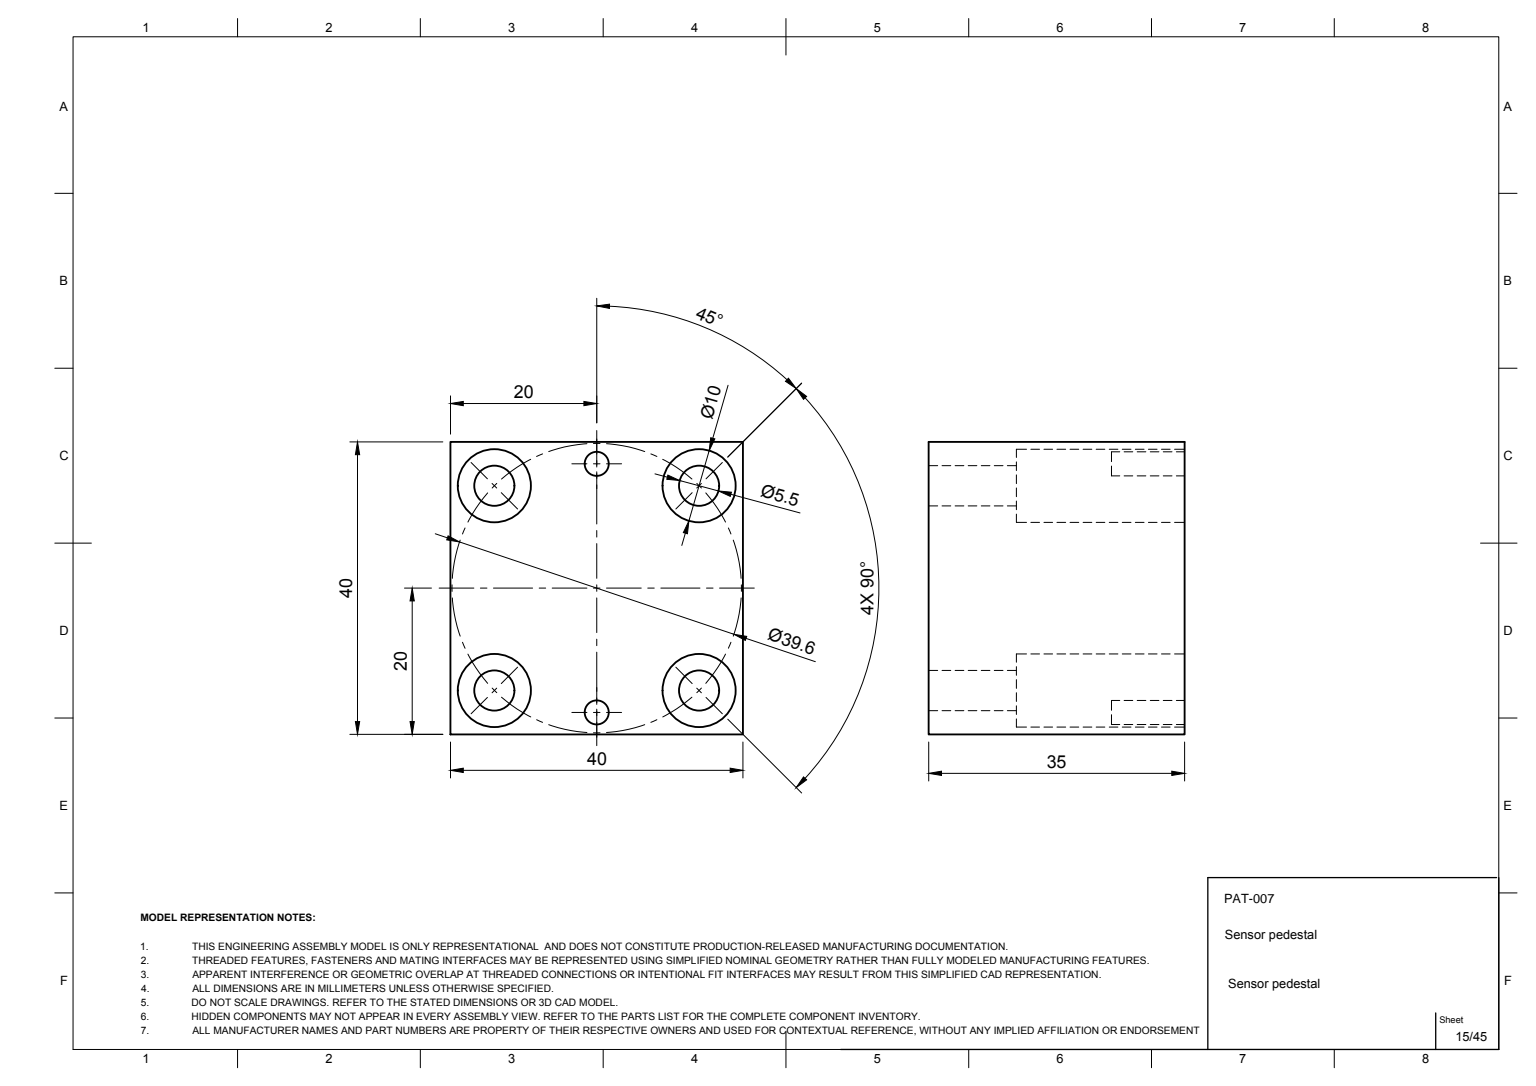
ISO-10303-21;
HEADER;
/* Generated by software containing ST-Developer
 * from STEP Tools, Inc. (www.steptools.com) 
 */

FILE_DESCRIPTION(
/* description */ ('Bearing friction torque test rig'),
/* implementation_level */ '2;1');

FILE_NAME(
/* name */ 'Sensor pedestal.step',
/* time_stamp */ '2026-10-28T03:24:04-07:00',
/* author */ (''),
/* organization */ (''),
/* preprocessor_version */ 'ST-DEVELOPER v20.2',
/* originating_system */ 'Autodesk Translation Framework v15.17.0.0',
/* authorisation */ '');

FILE_SCHEMA (('AUTOMOTIVE_DESIGN { 1 0 10303 214 3 1 1 }'));
ENDSEC;

DATA;
#10=MECHANICAL_DESIGN_GEOMETRIC_PRESENTATION_REPRESENTATION('',(#549),#14822);
#471=SHAPE_REPRESENTATION_RELATIONSHIP('SRR','None',#15010,#510);
#510=ADVANCED_BREP_SHAPE_REPRESENTATION('',(#603),#14790);
#549=STYLED_ITEM('',(#15298),#603);
#603=MANIFOLD_SOLID_BREP('Body1',#7665);
#777=FACE_BOUND('',#1816,.T.);
#778=FACE_BOUND('',#1819,.T.);
#779=FACE_BOUND('',#1822,.T.);
#780=FACE_BOUND('',#1825,.T.);
#781=FACE_BOUND('',#1835,.T.);
#782=FACE_BOUND('',#1836,.T.);
#783=FACE_BOUND('',#1837,.T.);
#784=FACE_BOUND('',#1838,.T.);
#785=FACE_BOUND('',#1839,.T.);
#786=FACE_BOUND('',#1840,.T.);
#787=FACE_BOUND('',#1842,.T.);
#788=FACE_BOUND('',#1843,.T.);
#789=FACE_BOUND('',#1844,.T.);
#790=FACE_BOUND('',#1845,.T.);
#927=PLANE('',#8461);
#928=PLANE('',#8465);
#929=PLANE('',#8469);
#930=PLANE('',#8474);
#931=PLANE('',#8479);
#932=PLANE('',#8484);
#933=PLANE('',#8494);
#934=PLANE('',#8495);
#935=PLANE('',#8496);
#936=PLANE('',#8497);
#937=PLANE('',#8498);
#938=PLANE('',#8499);
#1232=FACE_OUTER_BOUND('',#1810,.T.);
#1233=FACE_OUTER_BOUND('',#1811,.T.);
#1234=FACE_OUTER_BOUND('',#1812,.T.);
#1235=FACE_OUTER_BOUND('',#1813,.T.);
#1236=FACE_OUTER_BOUND('',#1814,.T.);
#1237=FACE_OUTER_BOUND('',#1815,.T.);
#1238=FACE_OUTER_BOUND('',#1817,.T.);
#1239=FACE_OUTER_BOUND('',#1818,.T.);
#1240=FACE_OUTER_BOUND('',#1820,.T.);
#1241=FACE_OUTER_BOUND('',#1821,.T.);
#1242=FACE_OUTER_BOUND('',#1823,.T.);
#1243=FACE_OUTER_BOUND('',#1824,.T.);
#1244=FACE_OUTER_BOUND('',#1826,.T.);
#1245=FACE_OUTER_BOUND('',#1827,.T.);
#1246=FACE_OUTER_BOUND('',#1828,.T.);
#1247=FACE_OUTER_BOUND('',#1829,.T.);
#1248=FACE_OUTER_BOUND('',#1830,.T.);
#1249=FACE_OUTER_BOUND('',#1831,.T.);
#1250=FACE_OUTER_BOUND('',#1832,.T.);
#1251=FACE_OUTER_BOUND('',#1833,.T.);
#1252=FACE_OUTER_BOUND('',#1834,.T.);
#1253=FACE_OUTER_BOUND('',#1841,.T.);
#1810=EDGE_LOOP('',(#5760,#5761,#5762,#5763));
#1811=EDGE_LOOP('',(#5764));
#1812=EDGE_LOOP('',(#5765,#5766,#5767,#5768));
#1813=EDGE_LOOP('',(#5769));
#1814=EDGE_LOOP('',(#5770,#5771,#5772,#5773));
#1815=EDGE_LOOP('',(#5774));
#1816=EDGE_LOOP('',(#5775));
#1817=EDGE_LOOP('',(#5776,#5777,#5778,#5779));
#1818=EDGE_LOOP('',(#5780));
#1819=EDGE_LOOP('',(#5781));
#1820=EDGE_LOOP('',(#5782,#5783,#5784,#5785));
#1821=EDGE_LOOP('',(#5786));
#1822=EDGE_LOOP('',(#5787));
#1823=EDGE_LOOP('',(#5788,#5789,#5790,#5791));
#1824=EDGE_LOOP('',(#5792));
#1825=EDGE_LOOP('',(#5793));
#1826=EDGE_LOOP('',(#5794,#5795,#5796,#5797));
#1827=EDGE_LOOP('',(#5798,#5799,#5800,#5801));
#1828=EDGE_LOOP('',(#5802,#5803,#5804,#5805));
#1829=EDGE_LOOP('',(#5806,#5807,#5808,#5809));
#1830=EDGE_LOOP('',(#5810,#5811,#5812,#5813));
#1831=EDGE_LOOP('',(#5814,#5815,#5816,#5817));
#1832=EDGE_LOOP('',(#5818,#5819,#5820,#5821));
#1833=EDGE_LOOP('',(#5822,#5823,#5824,#5825));
#1834=EDGE_LOOP('',(#5826,#5827,#5828,#5829));
#1835=EDGE_LOOP('',(#5830));
#1836=EDGE_LOOP('',(#5831));
#1837=EDGE_LOOP('',(#5832));
#1838=EDGE_LOOP('',(#5833));
#1839=EDGE_LOOP('',(#5834));
#1840=EDGE_LOOP('',(#5835));
#1841=EDGE_LOOP('',(#5836,#5837,#5838,#5839));
#1842=EDGE_LOOP('',(#5840));
#1843=EDGE_LOOP('',(#5841));
#1844=EDGE_LOOP('',(#5842));
#1845=EDGE_LOOP('',(#5843));
#2355=LINE('',#12318,#2799);
#2356=LINE('',#12325,#2800);
#2357=LINE('',#12332,#2801);
#2358=LINE('',#12341,#2802);
#2359=LINE('',#12350,#2803);
#2360=LINE('',#12359,#2804);
#2361=LINE('',#12367,#2805);
#2362=LINE('',#12371,#2806);
#2363=LINE('',#12375,#2807);
#2364=LINE('',#12379,#2808);
#2365=LINE('',#12383,#2809);
#2366=LINE('',#12385,#2810);
#2367=LINE('',#12387,#2811);
#2368=LINE('',#12388,#2812);
#2369=LINE('',#12391,#2813);
#2370=LINE('',#12393,#2814);
#2371=LINE('',#12394,#2815);
#2372=LINE('',#12397,#2816);
#2373=LINE('',#12399,#2817);
#2374=LINE('',#12400,#2818);
#2375=LINE('',#12402,#2819);
#2376=LINE('',#12403,#2820);
#2799=VECTOR('',#9938,0.164999999999999);
#2800=VECTOR('',#9947,0.164999999999999);
#2801=VECTOR('',#9956,0.5);
#2802=VECTOR('',#9967,0.5);
#2803=VECTOR('',#9978,0.5);
#2804=VECTOR('',#9989,0.5);
#2805=VECTOR('',#10000,0.275);
#2806=VECTOR('',#10005,0.275);
#2807=VECTOR('',#10010,0.275);
#2808=VECTOR('',#10015,0.275);
#2809=VECTOR('',#10018,1.);
#2810=VECTOR('',#10019,1.);
#2811=VECTOR('',#10020,1.);
#2812=VECTOR('',#10021,1.);
#2813=VECTOR('',#10024,1.);
#2814=VECTOR('',#10025,1.);
#2815=VECTOR('',#10026,1.);
#2816=VECTOR('',#10029,1.);
#2817=VECTOR('',#10030,1.);
#2818=VECTOR('',#10031,1.);
#2819=VECTOR('',#10034,1.);
#2820=VECTOR('',#10035,1.);
#3271=CIRCLE('',#8459,0.164999999999999);
#3272=CIRCLE('',#8460,0.164999999999999);
#3273=CIRCLE('',#8463,0.164999999999999);
#3274=CIRCLE('',#8464,0.164999999999999);
#3275=CIRCLE('',#8467,0.5);
#3276=CIRCLE('',#8468,0.5);
#3277=CIRCLE('',#8470,0.275);
#3278=CIRCLE('',#8472,0.5);
#3279=CIRCLE('',#8473,0.5);
#3280=CIRCLE('',#8475,0.275);
#3281=CIRCLE('',#8477,0.5);
#3282=CIRCLE('',#8478,0.5);
#3283=CIRCLE('',#8480,0.275);
#3284=CIRCLE('',#8482,0.5);
#3285=CIRCLE('',#8483,0.5);
#3286=CIRCLE('',#8485,0.275);
#3287=CIRCLE('',#8487,0.275);
#3288=CIRCLE('',#8489,0.275);
#3289=CIRCLE('',#8491,0.275);
#3290=CIRCLE('',#8493,0.275);
#3757=VERTEX_POINT('',#12315);
#3758=VERTEX_POINT('',#12317);
#3759=VERTEX_POINT('',#12322);
#3760=VERTEX_POINT('',#12324);
#3761=VERTEX_POINT('',#12329);
#3762=VERTEX_POINT('',#12331);
#3763=VERTEX_POINT('',#12335);
#3764=VERTEX_POINT('',#12338);
#3765=VERTEX_POINT('',#12340);
#3766=VERTEX_POINT('',#12344);
#3767=VERTEX_POINT('',#12347);
#3768=VERTEX_POINT('',#12349);
#3769=VERTEX_POINT('',#12353);
#3770=VERTEX_POINT('',#12356);
#3771=VERTEX_POINT('',#12358);
#3772=VERTEX_POINT('',#12362);
#3773=VERTEX_POINT('',#12365);
#3774=VERTEX_POINT('',#12369);
#3775=VERTEX_POINT('',#12373);
#3776=VERTEX_POINT('',#12377);
#3777=VERTEX_POINT('',#12381);
#3778=VERTEX_POINT('',#12382);
#3779=VERTEX_POINT('',#12384);
#3780=VERTEX_POINT('',#12386);
#3781=VERTEX_POINT('',#12390);
#3782=VERTEX_POINT('',#12392);
#3783=VERTEX_POINT('',#12396);
#3784=VERTEX_POINT('',#12398);
#4506=EDGE_CURVE('',#3757,#3757,#3271,.T.);
#4507=EDGE_CURVE('',#3757,#3758,#2355,.T.);
#4508=EDGE_CURVE('',#3758,#3758,#3272,.T.);
#4509=EDGE_CURVE('',#3759,#3759,#3273,.T.);
#4510=EDGE_CURVE('',#3759,#3760,#2356,.T.);
#4511=EDGE_CURVE('',#3760,#3760,#3274,.T.);
#4512=EDGE_CURVE('',#3761,#3761,#3275,.T.);
#4513=EDGE_CURVE('',#3761,#3762,#2357,.T.);
#4514=EDGE_CURVE('',#3762,#3762,#3276,.T.);
#4515=EDGE_CURVE('',#3763,#3763,#3277,.T.);
#4516=EDGE_CURVE('',#3764,#3764,#3278,.T.);
#4517=EDGE_CURVE('',#3764,#3765,#2358,.T.);
#4518=EDGE_CURVE('',#3765,#3765,#3279,.T.);
#4519=EDGE_CURVE('',#3766,#3766,#3280,.T.);
#4520=EDGE_CURVE('',#3767,#3767,#3281,.T.);
#4521=EDGE_CURVE('',#3767,#3768,#2359,.T.);
#4522=EDGE_CURVE('',#3768,#3768,#3282,.T.);
#4523=EDGE_CURVE('',#3769,#3769,#3283,.T.);
#4524=EDGE_CURVE('',#3770,#3770,#3284,.T.);
#4525=EDGE_CURVE('',#3770,#3771,#2360,.T.);
#4526=EDGE_CURVE('',#3771,#3771,#3285,.T.);
#4527=EDGE_CURVE('',#3772,#3772,#3286,.T.);
#4528=EDGE_CURVE('',#3773,#3773,#3287,.T.);
#4529=EDGE_CURVE('',#3773,#3763,#2361,.T.);
#4530=EDGE_CURVE('',#3774,#3774,#3288,.T.);
#4531=EDGE_CURVE('',#3774,#3766,#2362,.T.);
#4532=EDGE_CURVE('',#3775,#3775,#3289,.T.);
#4533=EDGE_CURVE('',#3775,#3769,#2363,.T.);
#4534=EDGE_CURVE('',#3776,#3776,#3290,.T.);
#4535=EDGE_CURVE('',#3776,#3772,#2364,.T.);
#4536=EDGE_CURVE('',#3777,#3778,#2365,.T.);
#4537=EDGE_CURVE('',#3778,#3779,#2366,.T.);
#4538=EDGE_CURVE('',#3780,#3779,#2367,.T.);
#4539=EDGE_CURVE('',#3777,#3780,#2368,.T.);
#4540=EDGE_CURVE('',#3781,#3777,#2369,.T.);
#4541=EDGE_CURVE('',#3782,#3780,#2370,.T.);
#4542=EDGE_CURVE('',#3781,#3782,#2371,.T.);
#4543=EDGE_CURVE('',#3783,#3781,#2372,.T.);
#4544=EDGE_CURVE('',#3784,#3782,#2373,.T.);
#4545=EDGE_CURVE('',#3783,#3784,#2374,.T.);
#4546=EDGE_CURVE('',#3778,#3783,#2375,.T.);
#4547=EDGE_CURVE('',#3779,#3784,#2376,.T.);
#5760=ORIENTED_EDGE('',*,*,#4506,.F.);
#5761=ORIENTED_EDGE('',*,*,#4507,.T.);
#5762=ORIENTED_EDGE('',*,*,#4508,.F.);
#5763=ORIENTED_EDGE('',*,*,#4507,.F.);
#5764=ORIENTED_EDGE('',*,*,#4506,.T.);
#5765=ORIENTED_EDGE('',*,*,#4509,.F.);
#5766=ORIENTED_EDGE('',*,*,#4510,.T.);
#5767=ORIENTED_EDGE('',*,*,#4511,.F.);
#5768=ORIENTED_EDGE('',*,*,#4510,.F.);
#5769=ORIENTED_EDGE('',*,*,#4509,.T.);
#5770=ORIENTED_EDGE('',*,*,#4512,.F.);
#5771=ORIENTED_EDGE('',*,*,#4513,.T.);
#5772=ORIENTED_EDGE('',*,*,#4514,.F.);
#5773=ORIENTED_EDGE('',*,*,#4513,.F.);
#5774=ORIENTED_EDGE('',*,*,#4512,.T.);
#5775=ORIENTED_EDGE('',*,*,#4515,.F.);
#5776=ORIENTED_EDGE('',*,*,#4516,.F.);
#5777=ORIENTED_EDGE('',*,*,#4517,.T.);
#5778=ORIENTED_EDGE('',*,*,#4518,.F.);
#5779=ORIENTED_EDGE('',*,*,#4517,.F.);
#5780=ORIENTED_EDGE('',*,*,#4516,.T.);
#5781=ORIENTED_EDGE('',*,*,#4519,.F.);
#5782=ORIENTED_EDGE('',*,*,#4520,.F.);
#5783=ORIENTED_EDGE('',*,*,#4521,.T.);
#5784=ORIENTED_EDGE('',*,*,#4522,.F.);
#5785=ORIENTED_EDGE('',*,*,#4521,.F.);
#5786=ORIENTED_EDGE('',*,*,#4520,.T.);
#5787=ORIENTED_EDGE('',*,*,#4523,.F.);
#5788=ORIENTED_EDGE('',*,*,#4524,.F.);
#5789=ORIENTED_EDGE('',*,*,#4525,.T.);
#5790=ORIENTED_EDGE('',*,*,#4526,.F.);
#5791=ORIENTED_EDGE('',*,*,#4525,.F.);
#5792=ORIENTED_EDGE('',*,*,#4524,.T.);
#5793=ORIENTED_EDGE('',*,*,#4527,.F.);
#5794=ORIENTED_EDGE('',*,*,#4528,.F.);
#5795=ORIENTED_EDGE('',*,*,#4529,.T.);
#5796=ORIENTED_EDGE('',*,*,#4515,.T.);
#5797=ORIENTED_EDGE('',*,*,#4529,.F.);
#5798=ORIENTED_EDGE('',*,*,#4530,.F.);
#5799=ORIENTED_EDGE('',*,*,#4531,.T.);
#5800=ORIENTED_EDGE('',*,*,#4519,.T.);
#5801=ORIENTED_EDGE('',*,*,#4531,.F.);
#5802=ORIENTED_EDGE('',*,*,#4532,.F.);
#5803=ORIENTED_EDGE('',*,*,#4533,.T.);
#5804=ORIENTED_EDGE('',*,*,#4523,.T.);
#5805=ORIENTED_EDGE('',*,*,#4533,.F.);
#5806=ORIENTED_EDGE('',*,*,#4534,.F.);
#5807=ORIENTED_EDGE('',*,*,#4535,.T.);
#5808=ORIENTED_EDGE('',*,*,#4527,.T.);
#5809=ORIENTED_EDGE('',*,*,#4535,.F.);
#5810=ORIENTED_EDGE('',*,*,#4536,.T.);
#5811=ORIENTED_EDGE('',*,*,#4537,.T.);
#5812=ORIENTED_EDGE('',*,*,#4538,.F.);
#5813=ORIENTED_EDGE('',*,*,#4539,.F.);
#5814=ORIENTED_EDGE('',*,*,#4540,.T.);
#5815=ORIENTED_EDGE('',*,*,#4539,.T.);
#5816=ORIENTED_EDGE('',*,*,#4541,.F.);
#5817=ORIENTED_EDGE('',*,*,#4542,.F.);
#5818=ORIENTED_EDGE('',*,*,#4543,.T.);
#5819=ORIENTED_EDGE('',*,*,#4542,.T.);
#5820=ORIENTED_EDGE('',*,*,#4544,.F.);
#5821=ORIENTED_EDGE('',*,*,#4545,.F.);
#5822=ORIENTED_EDGE('',*,*,#4546,.T.);
#5823=ORIENTED_EDGE('',*,*,#4545,.T.);
#5824=ORIENTED_EDGE('',*,*,#4547,.F.);
#5825=ORIENTED_EDGE('',*,*,#4537,.F.);
#5826=ORIENTED_EDGE('',*,*,#4547,.T.);
#5827=ORIENTED_EDGE('',*,*,#4544,.T.);
#5828=ORIENTED_EDGE('',*,*,#4541,.T.);
#5829=ORIENTED_EDGE('',*,*,#4538,.T.);
#5830=ORIENTED_EDGE('',*,*,#4508,.T.);
#5831=ORIENTED_EDGE('',*,*,#4511,.T.);
#5832=ORIENTED_EDGE('',*,*,#4526,.T.);
#5833=ORIENTED_EDGE('',*,*,#4522,.T.);
#5834=ORIENTED_EDGE('',*,*,#4518,.T.);
#5835=ORIENTED_EDGE('',*,*,#4514,.T.);
#5836=ORIENTED_EDGE('',*,*,#4546,.F.);
#5837=ORIENTED_EDGE('',*,*,#4536,.F.);
#5838=ORIENTED_EDGE('',*,*,#4540,.F.);
#5839=ORIENTED_EDGE('',*,*,#4543,.F.);
#5840=ORIENTED_EDGE('',*,*,#4528,.T.);
#5841=ORIENTED_EDGE('',*,*,#4530,.T.);
#5842=ORIENTED_EDGE('',*,*,#4532,.T.);
#5843=ORIENTED_EDGE('',*,*,#4534,.T.);
#7124=CYLINDRICAL_SURFACE('',#8458,0.164999999999999);
#7125=CYLINDRICAL_SURFACE('',#8462,0.164999999999999);
#7126=CYLINDRICAL_SURFACE('',#8466,0.5);
#7127=CYLINDRICAL_SURFACE('',#8471,0.5);
#7128=CYLINDRICAL_SURFACE('',#8476,0.5);
#7129=CYLINDRICAL_SURFACE('',#8481,0.5);
#7130=CYLINDRICAL_SURFACE('',#8486,0.275);
#7131=CYLINDRICAL_SURFACE('',#8488,0.275);
#7132=CYLINDRICAL_SURFACE('',#8490,0.275);
#7133=CYLINDRICAL_SURFACE('',#8492,0.275);
#7343=ADVANCED_FACE('',(#1232),#7124,.F.);
#7344=ADVANCED_FACE('',(#1233),#927,.T.);
#7345=ADVANCED_FACE('',(#1234),#7125,.F.);
#7346=ADVANCED_FACE('',(#1235),#928,.T.);
#7347=ADVANCED_FACE('',(#1236),#7126,.F.);
#7348=ADVANCED_FACE('',(#1237,#777),#929,.T.);
#7349=ADVANCED_FACE('',(#1238),#7127,.F.);
#7350=ADVANCED_FACE('',(#1239,#778),#930,.T.);
#7351=ADVANCED_FACE('',(#1240),#7128,.F.);
#7352=ADVANCED_FACE('',(#1241,#779),#931,.T.);
#7353=ADVANCED_FACE('',(#1242),#7129,.F.);
#7354=ADVANCED_FACE('',(#1243,#780),#932,.T.);
#7355=ADVANCED_FACE('',(#1244),#7130,.F.);
#7356=ADVANCED_FACE('',(#1245),#7131,.F.);
#7357=ADVANCED_FACE('',(#1246),#7132,.F.);
#7358=ADVANCED_FACE('',(#1247),#7133,.F.);
#7359=ADVANCED_FACE('',(#1248),#933,.T.);
#7360=ADVANCED_FACE('',(#1249),#934,.T.);
#7361=ADVANCED_FACE('',(#1250),#935,.T.);
#7362=ADVANCED_FACE('',(#1251),#936,.T.);
#7363=ADVANCED_FACE('',(#1252,#781,#782,#783,#784,#785,#786),#937,.T.);
#7364=ADVANCED_FACE('',(#1253,#787,#788,#789,#790),#938,.F.);
#7665=CLOSED_SHELL('',(#7343,#7344,#7345,#7346,#7347,#7348,#7349,#7350,
#7351,#7352,#7353,#7354,#7355,#7356,#7357,#7358,#7359,#7360,#7361,#7362,
#7363,#7364));
#8457=AXIS2_PLACEMENT_3D('',#12313,#9932,#9933);
#8458=AXIS2_PLACEMENT_3D('',#12314,#9934,#9935);
#8459=AXIS2_PLACEMENT_3D('',#12316,#9936,#9937);
#8460=AXIS2_PLACEMENT_3D('',#12319,#9939,#9940);
#8461=AXIS2_PLACEMENT_3D('',#12320,#9941,#9942);
#8462=AXIS2_PLACEMENT_3D('',#12321,#9943,#9944);
#8463=AXIS2_PLACEMENT_3D('',#12323,#9945,#9946);
#8464=AXIS2_PLACEMENT_3D('',#12326,#9948,#9949);
#8465=AXIS2_PLACEMENT_3D('',#12327,#9950,#9951);
#8466=AXIS2_PLACEMENT_3D('',#12328,#9952,#9953);
#8467=AXIS2_PLACEMENT_3D('',#12330,#9954,#9955);
#8468=AXIS2_PLACEMENT_3D('',#12333,#9957,#9958);
#8469=AXIS2_PLACEMENT_3D('',#12334,#9959,#9960);
#8470=AXIS2_PLACEMENT_3D('',#12336,#9961,#9962);
#8471=AXIS2_PLACEMENT_3D('',#12337,#9963,#9964);
#8472=AXIS2_PLACEMENT_3D('',#12339,#9965,#9966);
#8473=AXIS2_PLACEMENT_3D('',#12342,#9968,#9969);
#8474=AXIS2_PLACEMENT_3D('',#12343,#9970,#9971);
#8475=AXIS2_PLACEMENT_3D('',#12345,#9972,#9973);
#8476=AXIS2_PLACEMENT_3D('',#12346,#9974,#9975);
#8477=AXIS2_PLACEMENT_3D('',#12348,#9976,#9977);
#8478=AXIS2_PLACEMENT_3D('',#12351,#9979,#9980);
#8479=AXIS2_PLACEMENT_3D('',#12352,#9981,#9982);
#8480=AXIS2_PLACEMENT_3D('',#12354,#9983,#9984);
#8481=AXIS2_PLACEMENT_3D('',#12355,#9985,#9986);
#8482=AXIS2_PLACEMENT_3D('',#12357,#9987,#9988);
#8483=AXIS2_PLACEMENT_3D('',#12360,#9990,#9991);
#8484=AXIS2_PLACEMENT_3D('',#12361,#9992,#9993);
#8485=AXIS2_PLACEMENT_3D('',#12363,#9994,#9995);
#8486=AXIS2_PLACEMENT_3D('',#12364,#9996,#9997);
#8487=AXIS2_PLACEMENT_3D('',#12366,#9998,#9999);
#8488=AXIS2_PLACEMENT_3D('',#12368,#10001,#10002);
#8489=AXIS2_PLACEMENT_3D('',#12370,#10003,#10004);
#8490=AXIS2_PLACEMENT_3D('',#12372,#10006,#10007);
#8491=AXIS2_PLACEMENT_3D('',#12374,#10008,#10009);
#8492=AXIS2_PLACEMENT_3D('',#12376,#10011,#10012);
#8493=AXIS2_PLACEMENT_3D('',#12378,#10013,#10014);
#8494=AXIS2_PLACEMENT_3D('',#12380,#10016,#10017);
#8495=AXIS2_PLACEMENT_3D('',#12389,#10022,#10023);
#8496=AXIS2_PLACEMENT_3D('',#12395,#10027,#10028);
#8497=AXIS2_PLACEMENT_3D('',#12401,#10032,#10033);
#8498=AXIS2_PLACEMENT_3D('',#12404,#10036,#10037);
#8499=AXIS2_PLACEMENT_3D('',#12405,#10038,#10039);
#9932=DIRECTION('axis',(0.,0.,1.));
#9933=DIRECTION('refdir',(1.,0.,0.));
#9934=DIRECTION('center_axis',(0.,0.,1.));
#9935=DIRECTION('ref_axis',(1.,0.,0.));
#9936=DIRECTION('center_axis',(0.,0.,1.));
#9937=DIRECTION('ref_axis',(1.,0.,0.));
#9938=DIRECTION('',(0.,0.,1.));
#9939=DIRECTION('center_axis',(0.,0.,-1.));
#9940=DIRECTION('ref_axis',(1.,0.,0.));
#9941=DIRECTION('center_axis',(0.,0.,1.));
#9942=DIRECTION('ref_axis',(1.,0.,0.));
#9943=DIRECTION('center_axis',(0.,0.,1.));
#9944=DIRECTION('ref_axis',(1.,0.,0.));
#9945=DIRECTION('center_axis',(0.,0.,1.));
#9946=DIRECTION('ref_axis',(1.,0.,0.));
#9947=DIRECTION('',(0.,0.,1.));
#9948=DIRECTION('center_axis',(0.,0.,-1.));
#9949=DIRECTION('ref_axis',(1.,0.,0.));
#9950=DIRECTION('center_axis',(0.,0.,1.));
#9951=DIRECTION('ref_axis',(1.,0.,0.));
#9952=DIRECTION('center_axis',(0.,0.,1.));
#9953=DIRECTION('ref_axis',(1.,0.,0.));
#9954=DIRECTION('center_axis',(0.,0.,1.));
#9955=DIRECTION('ref_axis',(1.,0.,0.));
#9956=DIRECTION('',(0.,0.,1.));
#9957=DIRECTION('center_axis',(0.,0.,-1.));
#9958=DIRECTION('ref_axis',(1.,0.,0.));
#9959=DIRECTION('center_axis',(0.,0.,1.));
#9960=DIRECTION('ref_axis',(1.,0.,0.));
#9961=DIRECTION('center_axis',(0.,0.,1.));
#9962=DIRECTION('ref_axis',(1.,0.,0.));
#9963=DIRECTION('center_axis',(0.,0.,1.));
#9964=DIRECTION('ref_axis',(1.,0.,0.));
#9965=DIRECTION('center_axis',(0.,0.,1.));
#9966=DIRECTION('ref_axis',(1.,0.,0.));
#9967=DIRECTION('',(0.,0.,1.));
#9968=DIRECTION('center_axis',(0.,0.,-1.));
#9969=DIRECTION('ref_axis',(1.,0.,0.));
#9970=DIRECTION('center_axis',(0.,0.,1.));
#9971=DIRECTION('ref_axis',(1.,0.,0.));
#9972=DIRECTION('center_axis',(0.,0.,1.));
#9973=DIRECTION('ref_axis',(1.,0.,0.));
#9974=DIRECTION('center_axis',(0.,0.,1.));
#9975=DIRECTION('ref_axis',(1.,0.,0.));
#9976=DIRECTION('center_axis',(0.,0.,1.));
#9977=DIRECTION('ref_axis',(1.,0.,0.));
#9978=DIRECTION('',(0.,0.,1.));
#9979=DIRECTION('center_axis',(0.,0.,-1.));
#9980=DIRECTION('ref_axis',(1.,0.,0.));
#9981=DIRECTION('center_axis',(0.,0.,1.));
#9982=DIRECTION('ref_axis',(1.,0.,0.));
#9983=DIRECTION('center_axis',(0.,0.,1.));
#9984=DIRECTION('ref_axis',(1.,0.,0.));
#9985=DIRECTION('center_axis',(0.,0.,1.));
#9986=DIRECTION('ref_axis',(1.,0.,0.));
#9987=DIRECTION('center_axis',(0.,0.,1.));
#9988=DIRECTION('ref_axis',(1.,0.,0.));
#9989=DIRECTION('',(0.,0.,1.));
#9990=DIRECTION('center_axis',(0.,0.,-1.));
#9991=DIRECTION('ref_axis',(1.,0.,0.));
#9992=DIRECTION('center_axis',(0.,0.,1.));
#9993=DIRECTION('ref_axis',(1.,0.,0.));
#9994=DIRECTION('center_axis',(0.,0.,1.));
#9995=DIRECTION('ref_axis',(1.,0.,0.));
#9996=DIRECTION('center_axis',(0.,0.,1.));
#9997=DIRECTION('ref_axis',(1.,0.,0.));
#9998=DIRECTION('center_axis',(0.,0.,1.));
#9999=DIRECTION('ref_axis',(1.,0.,0.));
#10000=DIRECTION('',(0.,0.,1.));
#10001=DIRECTION('center_axis',(0.,0.,1.));
#10002=DIRECTION('ref_axis',(1.,0.,0.));
#10003=DIRECTION('center_axis',(0.,0.,1.));
#10004=DIRECTION('ref_axis',(1.,0.,0.));
#10005=DIRECTION('',(0.,0.,1.));
#10006=DIRECTION('center_axis',(0.,0.,1.));
#10007=DIRECTION('ref_axis',(1.,0.,0.));
#10008=DIRECTION('center_axis',(0.,0.,1.));
#10009=DIRECTION('ref_axis',(1.,0.,0.));
#10010=DIRECTION('',(0.,0.,1.));
#10011=DIRECTION('center_axis',(0.,0.,1.));
#10012=DIRECTION('ref_axis',(1.,0.,0.));
#10013=DIRECTION('center_axis',(0.,0.,1.));
#10014=DIRECTION('ref_axis',(1.,0.,0.));
#10015=DIRECTION('',(0.,0.,1.));
#10016=DIRECTION('center_axis',(0.,1.,0.));
#10017=DIRECTION('ref_axis',(-1.,0.,0.));
#10018=DIRECTION('',(-1.,0.,0.));
#10019=DIRECTION('',(0.,0.,1.));
#10020=DIRECTION('',(-1.,0.,0.));
#10021=DIRECTION('',(0.,0.,1.));
#10022=DIRECTION('center_axis',(1.,0.,0.));
#10023=DIRECTION('ref_axis',(0.,1.,0.));
#10024=DIRECTION('',(0.,1.,0.));
#10025=DIRECTION('',(0.,1.,0.));
#10026=DIRECTION('',(0.,0.,1.));
#10027=DIRECTION('center_axis',(0.,-1.,0.));
#10028=DIRECTION('ref_axis',(1.,0.,0.));
#10029=DIRECTION('',(1.,0.,0.));
#10030=DIRECTION('',(1.,0.,0.));
#10031=DIRECTION('',(0.,0.,1.));
#10032=DIRECTION('center_axis',(-1.,0.,0.));
#10033=DIRECTION('ref_axis',(0.,-1.,0.));
#10034=DIRECTION('',(0.,-1.,0.));
#10035=DIRECTION('',(0.,-1.,0.));
#10036=DIRECTION('center_axis',(0.,0.,1.));
#10037=DIRECTION('ref_axis',(1.,0.,0.));
#10038=DIRECTION('center_axis',(0.,0.,1.));
#10039=DIRECTION('ref_axis',(1.,0.,0.));
#12313=CARTESIAN_POINT('',(0.,0.,0.));
#12314=CARTESIAN_POINT('Origin',(10.,-1.7,3.5));
#12315=CARTESIAN_POINT('',(9.835,-1.7,3.5));
#12316=CARTESIAN_POINT('Origin',(10.,-1.7,3.5));
#12317=CARTESIAN_POINT('',(9.835,-1.7,4.5));
#12318=CARTESIAN_POINT('',(9.835,-1.7,3.5));
#12319=CARTESIAN_POINT('Origin',(10.,-1.7,4.5));
#12320=CARTESIAN_POINT('Origin',(10.,-1.7,3.5));
#12321=CARTESIAN_POINT('Origin',(10.,1.7,3.5));
#12322=CARTESIAN_POINT('',(9.835,1.7,3.5));
#12323=CARTESIAN_POINT('Origin',(10.,1.7,3.5));
#12324=CARTESIAN_POINT('',(9.835,1.7,4.5));
#12325=CARTESIAN_POINT('',(9.835,1.7,3.5));
#12326=CARTESIAN_POINT('Origin',(10.,1.7,4.5));
#12327=CARTESIAN_POINT('Origin',(10.,1.7,3.5));
#12328=CARTESIAN_POINT('Origin',(11.4,-1.4,2.2));
#12329=CARTESIAN_POINT('',(10.9,-1.4,2.2));
#12330=CARTESIAN_POINT('Origin',(11.4,-1.4,2.2));
#12331=CARTESIAN_POINT('',(10.9,-1.4,4.5));
#12332=CARTESIAN_POINT('',(10.9,-1.4,2.2));
#12333=CARTESIAN_POINT('Origin',(11.4,-1.4,4.5));
#12334=CARTESIAN_POINT('Origin',(11.4,-1.4,2.2));
#12335=CARTESIAN_POINT('',(11.125,-1.4,2.2));
#12336=CARTESIAN_POINT('Origin',(11.4,-1.4,2.2));
#12337=CARTESIAN_POINT('Origin',(8.6,1.4,2.2));
#12338=CARTESIAN_POINT('',(8.1,1.4,2.2));
#12339=CARTESIAN_POINT('Origin',(8.6,1.4,2.2));
#12340=CARTESIAN_POINT('',(8.1,1.4,4.5));
#12341=CARTESIAN_POINT('',(8.1,1.4,2.2));
#12342=CARTESIAN_POINT('Origin',(8.6,1.4,4.5));
#12343=CARTESIAN_POINT('Origin',(8.6,1.4,2.2));
#12344=CARTESIAN_POINT('',(8.325,1.4,2.2));
#12345=CARTESIAN_POINT('Origin',(8.6,1.4,2.2));
#12346=CARTESIAN_POINT('Origin',(8.6,-1.4,2.2));
#12347=CARTESIAN_POINT('',(8.1,-1.4,2.2));
#12348=CARTESIAN_POINT('Origin',(8.6,-1.4,2.2));
#12349=CARTESIAN_POINT('',(8.1,-1.4,4.5));
#12350=CARTESIAN_POINT('',(8.1,-1.4,2.2));
#12351=CARTESIAN_POINT('Origin',(8.6,-1.4,4.5));
#12352=CARTESIAN_POINT('Origin',(8.6,-1.4,2.2));
#12353=CARTESIAN_POINT('',(8.325,-1.4,2.2));
#12354=CARTESIAN_POINT('Origin',(8.6,-1.4,2.2));
#12355=CARTESIAN_POINT('Origin',(11.4,1.4,2.2));
#12356=CARTESIAN_POINT('',(10.9,1.4,2.2));
#12357=CARTESIAN_POINT('Origin',(11.4,1.4,2.2));
#12358=CARTESIAN_POINT('',(10.9,1.4,4.5));
#12359=CARTESIAN_POINT('',(10.9,1.4,2.2));
#12360=CARTESIAN_POINT('Origin',(11.4,1.4,4.5));
#12361=CARTESIAN_POINT('Origin',(11.4,1.4,2.2));
#12362=CARTESIAN_POINT('',(11.125,1.4,2.2));
#12363=CARTESIAN_POINT('Origin',(11.4,1.4,2.2));
#12364=CARTESIAN_POINT('Origin',(11.4,-1.4,0.9));
#12365=CARTESIAN_POINT('',(11.125,-1.4,1.));
#12366=CARTESIAN_POINT('Origin',(11.4,-1.4,1.));
#12367=CARTESIAN_POINT('',(11.125,-1.4,0.9));
#12368=CARTESIAN_POINT('Origin',(8.6,1.4,0.9));
#12369=CARTESIAN_POINT('',(8.325,1.4,1.));
#12370=CARTESIAN_POINT('Origin',(8.6,1.4,1.));
#12371=CARTESIAN_POINT('',(8.325,1.4,0.9));
#12372=CARTESIAN_POINT('Origin',(8.6,-1.4,0.9));
#12373=CARTESIAN_POINT('',(8.325,-1.4,1.));
#12374=CARTESIAN_POINT('Origin',(8.6,-1.4,1.));
#12375=CARTESIAN_POINT('',(8.325,-1.4,0.9));
#12376=CARTESIAN_POINT('Origin',(11.4,1.4,0.9));
#12377=CARTESIAN_POINT('',(11.125,1.4,1.));
#12378=CARTESIAN_POINT('Origin',(11.4,1.4,1.));
#12379=CARTESIAN_POINT('',(11.125,1.4,0.9));
#12380=CARTESIAN_POINT('Origin',(12.,2.,1.));
#12381=CARTESIAN_POINT('',(12.,2.,1.));
#12382=CARTESIAN_POINT('',(8.,2.,1.));
#12383=CARTESIAN_POINT('',(12.,2.,1.));
#12384=CARTESIAN_POINT('',(8.,2.,4.5));
#12385=CARTESIAN_POINT('',(8.,2.,1.));
#12386=CARTESIAN_POINT('',(12.,2.,4.5));
#12387=CARTESIAN_POINT('',(12.,2.,4.5));
#12388=CARTESIAN_POINT('',(12.,2.,1.));
#12389=CARTESIAN_POINT('Origin',(12.,-2.,1.));
#12390=CARTESIAN_POINT('',(12.,-2.,1.));
#12391=CARTESIAN_POINT('',(12.,-2.,1.));
#12392=CARTESIAN_POINT('',(12.,-2.,4.5));
#12393=CARTESIAN_POINT('',(12.,-2.,4.5));
#12394=CARTESIAN_POINT('',(12.,-2.,1.));
#12395=CARTESIAN_POINT('Origin',(8.,-2.,1.));
#12396=CARTESIAN_POINT('',(8.,-2.,1.));
#12397=CARTESIAN_POINT('',(8.,-2.,1.));
#12398=CARTESIAN_POINT('',(8.,-2.,4.5));
#12399=CARTESIAN_POINT('',(8.,-2.,4.5));
#12400=CARTESIAN_POINT('',(8.,-2.,1.));
#12401=CARTESIAN_POINT('Origin',(8.,2.,1.));
#12402=CARTESIAN_POINT('',(8.,2.,1.));
#12403=CARTESIAN_POINT('',(8.,2.,4.5));
#12404=CARTESIAN_POINT('Origin',(10.,0.,4.5));
#12405=CARTESIAN_POINT('Origin',(10.,0.,1.));
#14745=UNCERTAINTY_MEASURE_WITH_UNIT(LENGTH_MEASURE(0.001),#14823,
'DISTANCE_ACCURACY_VALUE',
'Maximum model space distance between geometric entities at asserted c
onnectivities');
#14777=UNCERTAINTY_MEASURE_WITH_UNIT(LENGTH_MEASURE(0.001),#14823,
'DISTANCE_ACCURACY_VALUE',
'Maximum model space distance between geometric entities at asserted c
onnectivities');
#14790=(
GEOMETRIC_REPRESENTATION_CONTEXT(3)
GLOBAL_UNCERTAINTY_ASSIGNED_CONTEXT((#14745))
GLOBAL_UNIT_ASSIGNED_CONTEXT((#14823,#14825,#14826))
REPRESENTATION_CONTEXT('','3D')
);
#14822=(
GEOMETRIC_REPRESENTATION_CONTEXT(3)
GLOBAL_UNCERTAINTY_ASSIGNED_CONTEXT((#14777))
GLOBAL_UNIT_ASSIGNED_CONTEXT((#14823,#14825,#14826))
REPRESENTATION_CONTEXT('','3D')
);
#14823=(
LENGTH_UNIT()
NAMED_UNIT(*)
SI_UNIT(.CENTI.,.METRE.)
);
#14825=(
NAMED_UNIT(*)
PLANE_ANGLE_UNIT()
SI_UNIT($,.RADIAN.)
);
#14826=(
NAMED_UNIT(*)
SI_UNIT($,.STERADIAN.)
SOLID_ANGLE_UNIT()
);
#14839=SHAPE_DEFINITION_REPRESENTATION(#14883,#15010);
#14883=PRODUCT_DEFINITION_SHAPE('',$,#15055);
#15010=SHAPE_REPRESENTATION('',(#8457),#14790);
#15042=PRODUCT_DEFINITION_CONTEXT('part definition',#15176,'design');
#15055=PRODUCT_DEFINITION('Sensor pedestal','Sensor pedestal',#15099,#15042);
#15099=PRODUCT_DEFINITION_FORMATION('',$,#15190);
#15176=APPLICATION_CONTEXT(
'Core Data for Automotive Mechanical Design Process');
#15177=PRODUCT_CONTEXT('part definition',#15176,'mechanical');
#15190=PRODUCT('Sensor pedestal','Sensor pedestal','Sensor pedestal',(#15177));
#15292=COLOUR_RGB('Off White',0.89,0.88,0.83);
#15293=FILL_AREA_STYLE_COLOUR('',#15292);
#15294=FILL_AREA_STYLE('',(#15293));
#15295=SURFACE_STYLE_FILL_AREA(#15294);
#15296=SURFACE_SIDE_STYLE('',(#15295));
#15297=SURFACE_STYLE_USAGE(.BOTH.,#15296);
#15298=PRESENTATION_STYLE_ASSIGNMENT((#15297));
ENDSEC;
END-ISO-10303-21;
